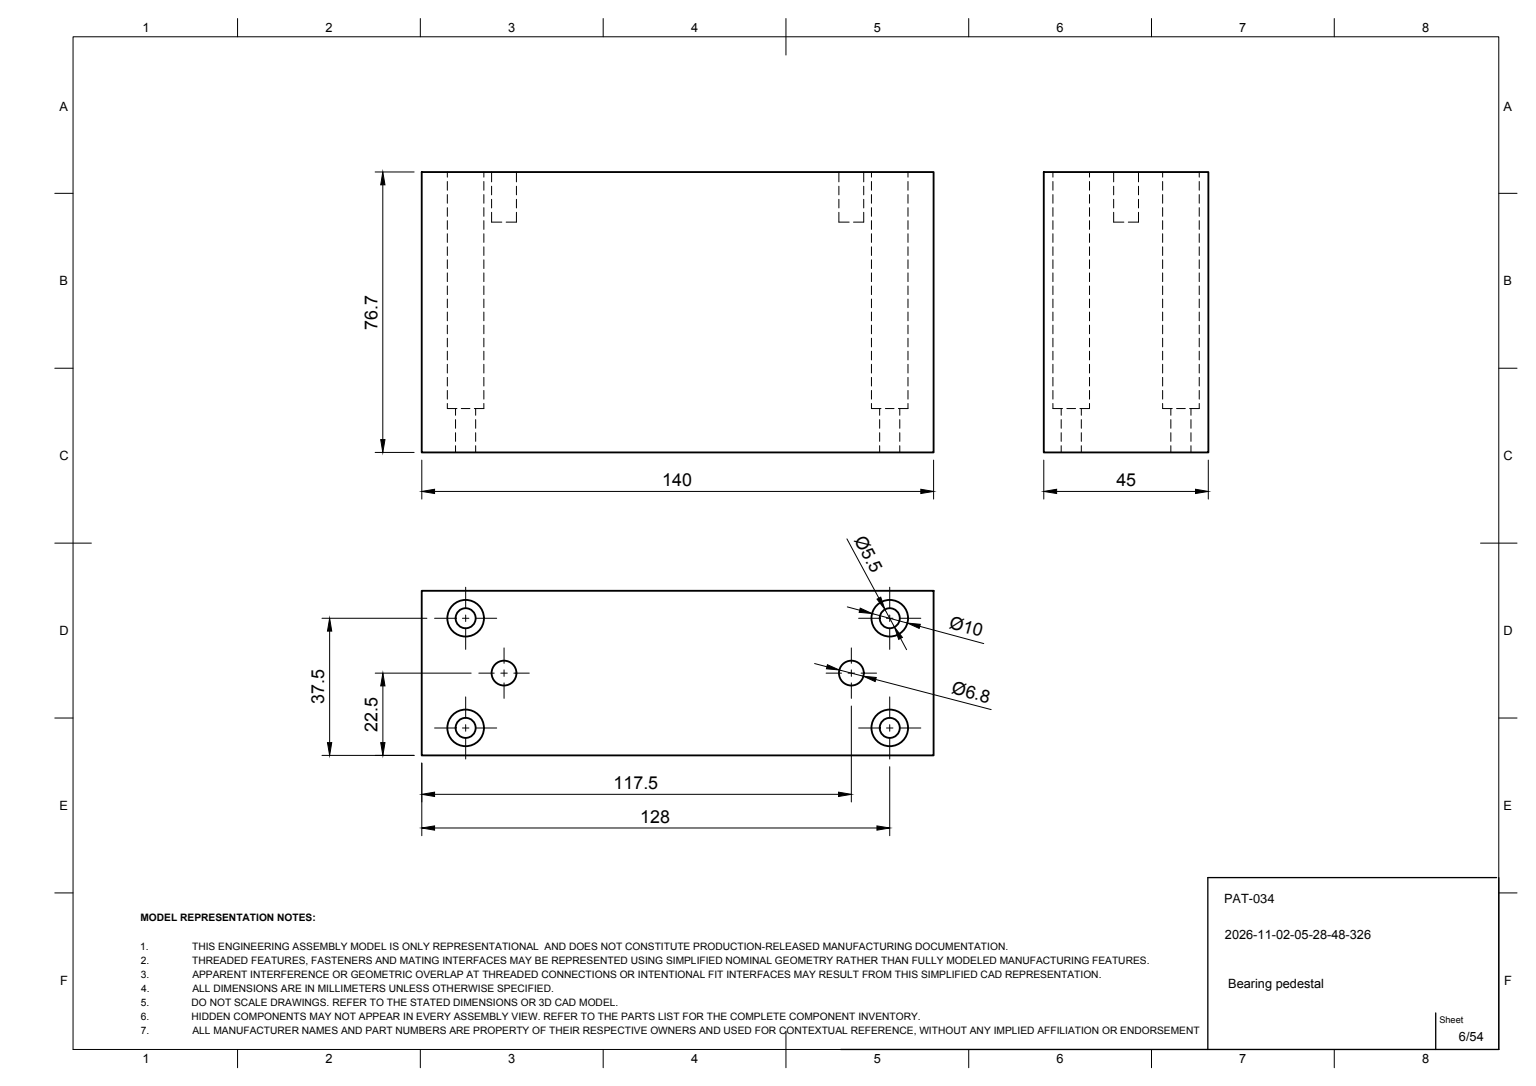
ISO-10303-21;
HEADER;
/* Generated by software containing ST-Developer
 * from STEP Tools, Inc. (www.steptools.com) 
 */

FILE_DESCRIPTION(
/* description */ ('Fatigue rig crank-slider'),
/* implementation_level */ '2;1');

FILE_NAME(
/* name */ 'Bearing pedestal.step',
/* time_stamp */ '2026-10-28T03:24:50-07:00',
/* author */ (''),
/* organization */ (''),
/* preprocessor_version */ 'ST-DEVELOPER v20.2',
/* originating_system */ 'Autodesk Translation Framework v15.17.0.0',
/* authorisation */ '');

FILE_SCHEMA (('AUTOMOTIVE_DESIGN { 1 0 10303 214 3 1 1 }'));
ENDSEC;

DATA;
#10=MECHANICAL_DESIGN_GEOMETRIC_PRESENTATION_REPRESENTATION('',(#588),#16911);
#488=SHAPE_REPRESENTATION_RELATIONSHIP('SRR','None',#17127,#538);
#538=ADVANCED_BREP_SHAPE_REPRESENTATION('',(#647),#16856);
#588=STYLED_ITEM('',(#17487),#647);
#647=MANIFOLD_SOLID_BREP('Body1',#8879);
#724=FACE_BOUND('',#1788,.T.);
#725=FACE_BOUND('',#1791,.T.);
#726=FACE_BOUND('',#1794,.T.);
#727=FACE_BOUND('',#1797,.T.);
#728=FACE_BOUND('',#1807,.T.);
#729=FACE_BOUND('',#1808,.T.);
#730=FACE_BOUND('',#1809,.T.);
#731=FACE_BOUND('',#1810,.T.);
#732=FACE_BOUND('',#1811,.T.);
#733=FACE_BOUND('',#1812,.T.);
#734=FACE_BOUND('',#1814,.T.);
#735=FACE_BOUND('',#1815,.T.);
#736=FACE_BOUND('',#1816,.T.);
#737=FACE_BOUND('',#1817,.T.);
#903=PLANE('',#9542);
#904=PLANE('',#9546);
#905=PLANE('',#9550);
#906=PLANE('',#9555);
#907=PLANE('',#9560);
#908=PLANE('',#9565);
#909=PLANE('',#9575);
#910=PLANE('',#9576);
#911=PLANE('',#9577);
#912=PLANE('',#9578);
#913=PLANE('',#9579);
#914=PLANE('',#9580);
#1235=FACE_OUTER_BOUND('',#1782,.T.);
#1236=FACE_OUTER_BOUND('',#1783,.T.);
#1237=FACE_OUTER_BOUND('',#1784,.T.);
#1238=FACE_OUTER_BOUND('',#1785,.T.);
#1239=FACE_OUTER_BOUND('',#1786,.T.);
#1240=FACE_OUTER_BOUND('',#1787,.T.);
#1241=FACE_OUTER_BOUND('',#1789,.T.);
#1242=FACE_OUTER_BOUND('',#1790,.T.);
#1243=FACE_OUTER_BOUND('',#1792,.T.);
#1244=FACE_OUTER_BOUND('',#1793,.T.);
#1245=FACE_OUTER_BOUND('',#1795,.T.);
#1246=FACE_OUTER_BOUND('',#1796,.T.);
#1247=FACE_OUTER_BOUND('',#1798,.T.);
#1248=FACE_OUTER_BOUND('',#1799,.T.);
#1249=FACE_OUTER_BOUND('',#1800,.T.);
#1250=FACE_OUTER_BOUND('',#1801,.T.);
#1251=FACE_OUTER_BOUND('',#1802,.T.);
#1252=FACE_OUTER_BOUND('',#1803,.T.);
#1253=FACE_OUTER_BOUND('',#1804,.T.);
#1254=FACE_OUTER_BOUND('',#1805,.T.);
#1255=FACE_OUTER_BOUND('',#1806,.T.);
#1256=FACE_OUTER_BOUND('',#1813,.T.);
#1782=EDGE_LOOP('',(#6092,#6093,#6094,#6095));
#1783=EDGE_LOOP('',(#6096));
#1784=EDGE_LOOP('',(#6097,#6098,#6099,#6100));
#1785=EDGE_LOOP('',(#6101));
#1786=EDGE_LOOP('',(#6102,#6103,#6104,#6105));
#1787=EDGE_LOOP('',(#6106));
#1788=EDGE_LOOP('',(#6107));
#1789=EDGE_LOOP('',(#6108,#6109,#6110,#6111));
#1790=EDGE_LOOP('',(#6112));
#1791=EDGE_LOOP('',(#6113));
#1792=EDGE_LOOP('',(#6114,#6115,#6116,#6117));
#1793=EDGE_LOOP('',(#6118));
#1794=EDGE_LOOP('',(#6119));
#1795=EDGE_LOOP('',(#6120,#6121,#6122,#6123));
#1796=EDGE_LOOP('',(#6124));
#1797=EDGE_LOOP('',(#6125));
#1798=EDGE_LOOP('',(#6126,#6127,#6128,#6129));
#1799=EDGE_LOOP('',(#6130,#6131,#6132,#6133));
#1800=EDGE_LOOP('',(#6134,#6135,#6136,#6137));
#1801=EDGE_LOOP('',(#6138,#6139,#6140,#6141));
#1802=EDGE_LOOP('',(#6142,#6143,#6144,#6145));
#1803=EDGE_LOOP('',(#6146,#6147,#6148,#6149));
#1804=EDGE_LOOP('',(#6150,#6151,#6152,#6153));
#1805=EDGE_LOOP('',(#6154,#6155,#6156,#6157));
#1806=EDGE_LOOP('',(#6158,#6159,#6160,#6161));
#1807=EDGE_LOOP('',(#6162));
#1808=EDGE_LOOP('',(#6163));
#1809=EDGE_LOOP('',(#6164));
#1810=EDGE_LOOP('',(#6165));
#1811=EDGE_LOOP('',(#6166));
#1812=EDGE_LOOP('',(#6167));
#1813=EDGE_LOOP('',(#6168,#6169,#6170,#6171));
#1814=EDGE_LOOP('',(#6172));
#1815=EDGE_LOOP('',(#6173));
#1816=EDGE_LOOP('',(#6174));
#1817=EDGE_LOOP('',(#6175));
#2484=LINE('',#13464,#3130);
#2485=LINE('',#13471,#3131);
#2486=LINE('',#13478,#3132);
#2487=LINE('',#13487,#3133);
#2488=LINE('',#13496,#3134);
#2489=LINE('',#13505,#3135);
#2490=LINE('',#13513,#3136);
#2491=LINE('',#13517,#3137);
#2492=LINE('',#13521,#3138);
#2493=LINE('',#13525,#3139);
#2494=LINE('',#13529,#3140);
#2495=LINE('',#13531,#3141);
#2496=LINE('',#13533,#3142);
#2497=LINE('',#13534,#3143);
#2498=LINE('',#13537,#3144);
#2499=LINE('',#13539,#3145);
#2500=LINE('',#13540,#3146);
#2501=LINE('',#13543,#3147);
#2502=LINE('',#13545,#3148);
#2503=LINE('',#13546,#3149);
#2504=LINE('',#13548,#3150);
#2505=LINE('',#13549,#3151);
#3130=VECTOR('',#10686,0.34);
#3131=VECTOR('',#10695,0.34);
#3132=VECTOR('',#10704,0.5);
#3133=VECTOR('',#10715,0.5);
#3134=VECTOR('',#10726,0.5);
#3135=VECTOR('',#10737,0.5);
#3136=VECTOR('',#10748,0.275);
#3137=VECTOR('',#10753,0.275);
#3138=VECTOR('',#10758,0.275);
#3139=VECTOR('',#10763,0.275);
#3140=VECTOR('',#10766,1.);
#3141=VECTOR('',#10767,1.);
#3142=VECTOR('',#10768,1.);
#3143=VECTOR('',#10769,1.);
#3144=VECTOR('',#10772,1.);
#3145=VECTOR('',#10773,1.);
#3146=VECTOR('',#10774,1.);
#3147=VECTOR('',#10777,1.);
#3148=VECTOR('',#10778,1.);
#3149=VECTOR('',#10779,1.);
#3150=VECTOR('',#10782,1.);
#3151=VECTOR('',#10783,1.);
#3776=CIRCLE('',#9540,0.34);
#3777=CIRCLE('',#9541,0.34);
#3778=CIRCLE('',#9544,0.34);
#3779=CIRCLE('',#9545,0.34);
#3780=CIRCLE('',#9548,0.5);
#3781=CIRCLE('',#9549,0.5);
#3782=CIRCLE('',#9551,0.275);
#3783=CIRCLE('',#9553,0.5);
#3784=CIRCLE('',#9554,0.5);
#3785=CIRCLE('',#9556,0.275);
#3786=CIRCLE('',#9558,0.5);
#3787=CIRCLE('',#9559,0.5);
#3788=CIRCLE('',#9561,0.275);
#3789=CIRCLE('',#9563,0.5);
#3790=CIRCLE('',#9564,0.5);
#3791=CIRCLE('',#9566,0.275);
#3792=CIRCLE('',#9568,0.275);
#3793=CIRCLE('',#9570,0.275);
#3794=CIRCLE('',#9572,0.275);
#3795=CIRCLE('',#9574,0.275);
#4184=VERTEX_POINT('',#13461);
#4185=VERTEX_POINT('',#13463);
#4186=VERTEX_POINT('',#13468);
#4187=VERTEX_POINT('',#13470);
#4188=VERTEX_POINT('',#13475);
#4189=VERTEX_POINT('',#13477);
#4190=VERTEX_POINT('',#13481);
#4191=VERTEX_POINT('',#13484);
#4192=VERTEX_POINT('',#13486);
#4193=VERTEX_POINT('',#13490);
#4194=VERTEX_POINT('',#13493);
#4195=VERTEX_POINT('',#13495);
#4196=VERTEX_POINT('',#13499);
#4197=VERTEX_POINT('',#13502);
#4198=VERTEX_POINT('',#13504);
#4199=VERTEX_POINT('',#13508);
#4200=VERTEX_POINT('',#13511);
#4201=VERTEX_POINT('',#13515);
#4202=VERTEX_POINT('',#13519);
#4203=VERTEX_POINT('',#13523);
#4204=VERTEX_POINT('',#13527);
#4205=VERTEX_POINT('',#13528);
#4206=VERTEX_POINT('',#13530);
#4207=VERTEX_POINT('',#13532);
#4208=VERTEX_POINT('',#13536);
#4209=VERTEX_POINT('',#13538);
#4210=VERTEX_POINT('',#13542);
#4211=VERTEX_POINT('',#13544);
#4944=EDGE_CURVE('',#4184,#4184,#3776,.T.);
#4945=EDGE_CURVE('',#4184,#4185,#2484,.T.);
#4946=EDGE_CURVE('',#4185,#4185,#3777,.T.);
#4947=EDGE_CURVE('',#4186,#4186,#3778,.T.);
#4948=EDGE_CURVE('',#4186,#4187,#2485,.T.);
#4949=EDGE_CURVE('',#4187,#4187,#3779,.T.);
#4950=EDGE_CURVE('',#4188,#4188,#3780,.T.);
#4951=EDGE_CURVE('',#4188,#4189,#2486,.T.);
#4952=EDGE_CURVE('',#4189,#4189,#3781,.T.);
#4953=EDGE_CURVE('',#4190,#4190,#3782,.T.);
#4954=EDGE_CURVE('',#4191,#4191,#3783,.T.);
#4955=EDGE_CURVE('',#4191,#4192,#2487,.T.);
#4956=EDGE_CURVE('',#4192,#4192,#3784,.T.);
#4957=EDGE_CURVE('',#4193,#4193,#3785,.T.);
#4958=EDGE_CURVE('',#4194,#4194,#3786,.T.);
#4959=EDGE_CURVE('',#4194,#4195,#2488,.T.);
#4960=EDGE_CURVE('',#4195,#4195,#3787,.T.);
#4961=EDGE_CURVE('',#4196,#4196,#3788,.T.);
#4962=EDGE_CURVE('',#4197,#4197,#3789,.T.);
#4963=EDGE_CURVE('',#4197,#4198,#2489,.T.);
#4964=EDGE_CURVE('',#4198,#4198,#3790,.T.);
#4965=EDGE_CURVE('',#4199,#4199,#3791,.T.);
#4966=EDGE_CURVE('',#4200,#4200,#3792,.T.);
#4967=EDGE_CURVE('',#4200,#4190,#2490,.T.);
#4968=EDGE_CURVE('',#4201,#4201,#3793,.T.);
#4969=EDGE_CURVE('',#4201,#4193,#2491,.T.);
#4970=EDGE_CURVE('',#4202,#4202,#3794,.T.);
#4971=EDGE_CURVE('',#4202,#4196,#2492,.T.);
#4972=EDGE_CURVE('',#4203,#4203,#3795,.T.);
#4973=EDGE_CURVE('',#4203,#4199,#2493,.T.);
#4974=EDGE_CURVE('',#4204,#4205,#2494,.T.);
#4975=EDGE_CURVE('',#4205,#4206,#2495,.T.);
#4976=EDGE_CURVE('',#4207,#4206,#2496,.T.);
#4977=EDGE_CURVE('',#4204,#4207,#2497,.T.);
#4978=EDGE_CURVE('',#4208,#4204,#2498,.T.);
#4979=EDGE_CURVE('',#4209,#4207,#2499,.T.);
#4980=EDGE_CURVE('',#4208,#4209,#2500,.T.);
#4981=EDGE_CURVE('',#4210,#4208,#2501,.T.);
#4982=EDGE_CURVE('',#4211,#4209,#2502,.T.);
#4983=EDGE_CURVE('',#4210,#4211,#2503,.T.);
#4984=EDGE_CURVE('',#4205,#4210,#2504,.T.);
#4985=EDGE_CURVE('',#4206,#4211,#2505,.T.);
#6092=ORIENTED_EDGE('',*,*,#4944,.F.);
#6093=ORIENTED_EDGE('',*,*,#4945,.T.);
#6094=ORIENTED_EDGE('',*,*,#4946,.F.);
#6095=ORIENTED_EDGE('',*,*,#4945,.F.);
#6096=ORIENTED_EDGE('',*,*,#4944,.T.);
#6097=ORIENTED_EDGE('',*,*,#4947,.F.);
#6098=ORIENTED_EDGE('',*,*,#4948,.T.);
#6099=ORIENTED_EDGE('',*,*,#4949,.F.);
#6100=ORIENTED_EDGE('',*,*,#4948,.F.);
#6101=ORIENTED_EDGE('',*,*,#4947,.T.);
#6102=ORIENTED_EDGE('',*,*,#4950,.F.);
#6103=ORIENTED_EDGE('',*,*,#4951,.T.);
#6104=ORIENTED_EDGE('',*,*,#4952,.F.);
#6105=ORIENTED_EDGE('',*,*,#4951,.F.);
#6106=ORIENTED_EDGE('',*,*,#4950,.T.);
#6107=ORIENTED_EDGE('',*,*,#4953,.F.);
#6108=ORIENTED_EDGE('',*,*,#4954,.F.);
#6109=ORIENTED_EDGE('',*,*,#4955,.T.);
#6110=ORIENTED_EDGE('',*,*,#4956,.F.);
#6111=ORIENTED_EDGE('',*,*,#4955,.F.);
#6112=ORIENTED_EDGE('',*,*,#4954,.T.);
#6113=ORIENTED_EDGE('',*,*,#4957,.F.);
#6114=ORIENTED_EDGE('',*,*,#4958,.F.);
#6115=ORIENTED_EDGE('',*,*,#4959,.T.);
#6116=ORIENTED_EDGE('',*,*,#4960,.F.);
#6117=ORIENTED_EDGE('',*,*,#4959,.F.);
#6118=ORIENTED_EDGE('',*,*,#4958,.T.);
#6119=ORIENTED_EDGE('',*,*,#4961,.F.);
#6120=ORIENTED_EDGE('',*,*,#4962,.F.);
#6121=ORIENTED_EDGE('',*,*,#4963,.T.);
#6122=ORIENTED_EDGE('',*,*,#4964,.F.);
#6123=ORIENTED_EDGE('',*,*,#4963,.F.);
#6124=ORIENTED_EDGE('',*,*,#4962,.T.);
#6125=ORIENTED_EDGE('',*,*,#4965,.F.);
#6126=ORIENTED_EDGE('',*,*,#4966,.F.);
#6127=ORIENTED_EDGE('',*,*,#4967,.T.);
#6128=ORIENTED_EDGE('',*,*,#4953,.T.);
#6129=ORIENTED_EDGE('',*,*,#4967,.F.);
#6130=ORIENTED_EDGE('',*,*,#4968,.F.);
#6131=ORIENTED_EDGE('',*,*,#4969,.T.);
#6132=ORIENTED_EDGE('',*,*,#4957,.T.);
#6133=ORIENTED_EDGE('',*,*,#4969,.F.);
#6134=ORIENTED_EDGE('',*,*,#4970,.F.);
#6135=ORIENTED_EDGE('',*,*,#4971,.T.);
#6136=ORIENTED_EDGE('',*,*,#4961,.T.);
#6137=ORIENTED_EDGE('',*,*,#4971,.F.);
#6138=ORIENTED_EDGE('',*,*,#4972,.F.);
#6139=ORIENTED_EDGE('',*,*,#4973,.T.);
#6140=ORIENTED_EDGE('',*,*,#4965,.T.);
#6141=ORIENTED_EDGE('',*,*,#4973,.F.);
#6142=ORIENTED_EDGE('',*,*,#4974,.T.);
#6143=ORIENTED_EDGE('',*,*,#4975,.T.);
#6144=ORIENTED_EDGE('',*,*,#4976,.F.);
#6145=ORIENTED_EDGE('',*,*,#4977,.F.);
#6146=ORIENTED_EDGE('',*,*,#4978,.T.);
#6147=ORIENTED_EDGE('',*,*,#4977,.T.);
#6148=ORIENTED_EDGE('',*,*,#4979,.F.);
#6149=ORIENTED_EDGE('',*,*,#4980,.F.);
#6150=ORIENTED_EDGE('',*,*,#4981,.T.);
#6151=ORIENTED_EDGE('',*,*,#4980,.T.);
#6152=ORIENTED_EDGE('',*,*,#4982,.F.);
#6153=ORIENTED_EDGE('',*,*,#4983,.F.);
#6154=ORIENTED_EDGE('',*,*,#4984,.T.);
#6155=ORIENTED_EDGE('',*,*,#4983,.T.);
#6156=ORIENTED_EDGE('',*,*,#4985,.F.);
#6157=ORIENTED_EDGE('',*,*,#4975,.F.);
#6158=ORIENTED_EDGE('',*,*,#4985,.T.);
#6159=ORIENTED_EDGE('',*,*,#4982,.T.);
#6160=ORIENTED_EDGE('',*,*,#4979,.T.);
#6161=ORIENTED_EDGE('',*,*,#4976,.T.);
#6162=ORIENTED_EDGE('',*,*,#4946,.T.);
#6163=ORIENTED_EDGE('',*,*,#4949,.T.);
#6164=ORIENTED_EDGE('',*,*,#4964,.T.);
#6165=ORIENTED_EDGE('',*,*,#4960,.T.);
#6166=ORIENTED_EDGE('',*,*,#4956,.T.);
#6167=ORIENTED_EDGE('',*,*,#4952,.T.);
#6168=ORIENTED_EDGE('',*,*,#4984,.F.);
#6169=ORIENTED_EDGE('',*,*,#4974,.F.);
#6170=ORIENTED_EDGE('',*,*,#4978,.F.);
#6171=ORIENTED_EDGE('',*,*,#4981,.F.);
#6172=ORIENTED_EDGE('',*,*,#4966,.T.);
#6173=ORIENTED_EDGE('',*,*,#4968,.T.);
#6174=ORIENTED_EDGE('',*,*,#4970,.T.);
#6175=ORIENTED_EDGE('',*,*,#4972,.T.);
#8208=CYLINDRICAL_SURFACE('',#9539,0.34);
#8209=CYLINDRICAL_SURFACE('',#9543,0.34);
#8210=CYLINDRICAL_SURFACE('',#9547,0.5);
#8211=CYLINDRICAL_SURFACE('',#9552,0.5);
#8212=CYLINDRICAL_SURFACE('',#9557,0.5);
#8213=CYLINDRICAL_SURFACE('',#9562,0.5);
#8214=CYLINDRICAL_SURFACE('',#9567,0.275);
#8215=CYLINDRICAL_SURFACE('',#9569,0.275);
#8216=CYLINDRICAL_SURFACE('',#9571,0.275);
#8217=CYLINDRICAL_SURFACE('',#9573,0.275);
#8373=ADVANCED_FACE('',(#1235),#8208,.F.);
#8374=ADVANCED_FACE('',(#1236),#903,.T.);
#8375=ADVANCED_FACE('',(#1237),#8209,.F.);
#8376=ADVANCED_FACE('',(#1238),#904,.T.);
#8377=ADVANCED_FACE('',(#1239),#8210,.F.);
#8378=ADVANCED_FACE('',(#1240,#724),#905,.T.);
#8379=ADVANCED_FACE('',(#1241),#8211,.F.);
#8380=ADVANCED_FACE('',(#1242,#725),#906,.T.);
#8381=ADVANCED_FACE('',(#1243),#8212,.F.);
#8382=ADVANCED_FACE('',(#1244,#726),#907,.T.);
#8383=ADVANCED_FACE('',(#1245),#8213,.F.);
#8384=ADVANCED_FACE('',(#1246,#727),#908,.T.);
#8385=ADVANCED_FACE('',(#1247),#8214,.F.);
#8386=ADVANCED_FACE('',(#1248),#8215,.F.);
#8387=ADVANCED_FACE('',(#1249),#8216,.F.);
#8388=ADVANCED_FACE('',(#1250),#8217,.F.);
#8389=ADVANCED_FACE('',(#1251),#909,.T.);
#8390=ADVANCED_FACE('',(#1252),#910,.T.);
#8391=ADVANCED_FACE('',(#1253),#911,.T.);
#8392=ADVANCED_FACE('',(#1254),#912,.T.);
#8393=ADVANCED_FACE('',(#1255,#728,#729,#730,#731,#732,#733),#913,.T.);
#8394=ADVANCED_FACE('',(#1256,#734,#735,#736,#737),#914,.F.);
#8879=CLOSED_SHELL('',(#8373,#8374,#8375,#8376,#8377,#8378,#8379,#8380,
#8381,#8382,#8383,#8384,#8385,#8386,#8387,#8388,#8389,#8390,#8391,#8392,
#8393,#8394));
#9538=AXIS2_PLACEMENT_3D('',#13459,#10680,#10681);
#9539=AXIS2_PLACEMENT_3D('',#13460,#10682,#10683);
#9540=AXIS2_PLACEMENT_3D('',#13462,#10684,#10685);
#9541=AXIS2_PLACEMENT_3D('',#13465,#10687,#10688);
#9542=AXIS2_PLACEMENT_3D('',#13466,#10689,#10690);
#9543=AXIS2_PLACEMENT_3D('',#13467,#10691,#10692);
#9544=AXIS2_PLACEMENT_3D('',#13469,#10693,#10694);
#9545=AXIS2_PLACEMENT_3D('',#13472,#10696,#10697);
#9546=AXIS2_PLACEMENT_3D('',#13473,#10698,#10699);
#9547=AXIS2_PLACEMENT_3D('',#13474,#10700,#10701);
#9548=AXIS2_PLACEMENT_3D('',#13476,#10702,#10703);
#9549=AXIS2_PLACEMENT_3D('',#13479,#10705,#10706);
#9550=AXIS2_PLACEMENT_3D('',#13480,#10707,#10708);
#9551=AXIS2_PLACEMENT_3D('',#13482,#10709,#10710);
#9552=AXIS2_PLACEMENT_3D('',#13483,#10711,#10712);
#9553=AXIS2_PLACEMENT_3D('',#13485,#10713,#10714);
#9554=AXIS2_PLACEMENT_3D('',#13488,#10716,#10717);
#9555=AXIS2_PLACEMENT_3D('',#13489,#10718,#10719);
#9556=AXIS2_PLACEMENT_3D('',#13491,#10720,#10721);
#9557=AXIS2_PLACEMENT_3D('',#13492,#10722,#10723);
#9558=AXIS2_PLACEMENT_3D('',#13494,#10724,#10725);
#9559=AXIS2_PLACEMENT_3D('',#13497,#10727,#10728);
#9560=AXIS2_PLACEMENT_3D('',#13498,#10729,#10730);
#9561=AXIS2_PLACEMENT_3D('',#13500,#10731,#10732);
#9562=AXIS2_PLACEMENT_3D('',#13501,#10733,#10734);
#9563=AXIS2_PLACEMENT_3D('',#13503,#10735,#10736);
#9564=AXIS2_PLACEMENT_3D('',#13506,#10738,#10739);
#9565=AXIS2_PLACEMENT_3D('',#13507,#10740,#10741);
#9566=AXIS2_PLACEMENT_3D('',#13509,#10742,#10743);
#9567=AXIS2_PLACEMENT_3D('',#13510,#10744,#10745);
#9568=AXIS2_PLACEMENT_3D('',#13512,#10746,#10747);
#9569=AXIS2_PLACEMENT_3D('',#13514,#10749,#10750);
#9570=AXIS2_PLACEMENT_3D('',#13516,#10751,#10752);
#9571=AXIS2_PLACEMENT_3D('',#13518,#10754,#10755);
#9572=AXIS2_PLACEMENT_3D('',#13520,#10756,#10757);
#9573=AXIS2_PLACEMENT_3D('',#13522,#10759,#10760);
#9574=AXIS2_PLACEMENT_3D('',#13524,#10761,#10762);
#9575=AXIS2_PLACEMENT_3D('',#13526,#10764,#10765);
#9576=AXIS2_PLACEMENT_3D('',#13535,#10770,#10771);
#9577=AXIS2_PLACEMENT_3D('',#13541,#10775,#10776);
#9578=AXIS2_PLACEMENT_3D('',#13547,#10780,#10781);
#9579=AXIS2_PLACEMENT_3D('',#13550,#10784,#10785);
#9580=AXIS2_PLACEMENT_3D('',#13551,#10786,#10787);
#10680=DIRECTION('axis',(0.,0.,1.));
#10681=DIRECTION('refdir',(1.,0.,0.));
#10682=DIRECTION('center_axis',(0.,0.,1.));
#10683=DIRECTION('ref_axis',(1.,0.,0.));
#10684=DIRECTION('center_axis',(0.,0.,1.));
#10685=DIRECTION('ref_axis',(1.,0.,0.));
#10686=DIRECTION('',(0.,0.,1.));
#10687=DIRECTION('center_axis',(0.,0.,-1.));
#10688=DIRECTION('ref_axis',(1.,0.,0.));
#10689=DIRECTION('center_axis',(0.,0.,1.));
#10690=DIRECTION('ref_axis',(1.,0.,0.));
#10691=DIRECTION('center_axis',(0.,0.,1.));
#10692=DIRECTION('ref_axis',(1.,0.,0.));
#10693=DIRECTION('center_axis',(0.,0.,1.));
#10694=DIRECTION('ref_axis',(1.,0.,0.));
#10695=DIRECTION('',(0.,0.,1.));
#10696=DIRECTION('center_axis',(0.,0.,-1.));
#10697=DIRECTION('ref_axis',(1.,0.,0.));
#10698=DIRECTION('center_axis',(0.,0.,1.));
#10699=DIRECTION('ref_axis',(1.,0.,0.));
#10700=DIRECTION('center_axis',(0.,0.,1.));
#10701=DIRECTION('ref_axis',(1.,0.,0.));
#10702=DIRECTION('center_axis',(0.,0.,1.));
#10703=DIRECTION('ref_axis',(1.,0.,0.));
#10704=DIRECTION('',(0.,0.,1.));
#10705=DIRECTION('center_axis',(0.,0.,-1.));
#10706=DIRECTION('ref_axis',(1.,0.,0.));
#10707=DIRECTION('center_axis',(0.,0.,1.));
#10708=DIRECTION('ref_axis',(1.,0.,0.));
#10709=DIRECTION('center_axis',(0.,0.,1.));
#10710=DIRECTION('ref_axis',(1.,0.,0.));
#10711=DIRECTION('center_axis',(0.,0.,1.));
#10712=DIRECTION('ref_axis',(1.,0.,0.));
#10713=DIRECTION('center_axis',(0.,0.,1.));
#10714=DIRECTION('ref_axis',(1.,0.,0.));
#10715=DIRECTION('',(0.,0.,1.));
#10716=DIRECTION('center_axis',(0.,0.,-1.));
#10717=DIRECTION('ref_axis',(1.,0.,0.));
#10718=DIRECTION('center_axis',(0.,0.,1.));
#10719=DIRECTION('ref_axis',(1.,0.,0.));
#10720=DIRECTION('center_axis',(0.,0.,1.));
#10721=DIRECTION('ref_axis',(1.,0.,0.));
#10722=DIRECTION('center_axis',(0.,0.,1.));
#10723=DIRECTION('ref_axis',(1.,0.,0.));
#10724=DIRECTION('center_axis',(0.,0.,1.));
#10725=DIRECTION('ref_axis',(1.,0.,0.));
#10726=DIRECTION('',(0.,0.,1.));
#10727=DIRECTION('center_axis',(0.,0.,-1.));
#10728=DIRECTION('ref_axis',(1.,0.,0.));
#10729=DIRECTION('center_axis',(0.,0.,1.));
#10730=DIRECTION('ref_axis',(1.,0.,0.));
#10731=DIRECTION('center_axis',(0.,0.,1.));
#10732=DIRECTION('ref_axis',(1.,0.,0.));
#10733=DIRECTION('center_axis',(0.,0.,1.));
#10734=DIRECTION('ref_axis',(1.,0.,0.));
#10735=DIRECTION('center_axis',(0.,0.,1.));
#10736=DIRECTION('ref_axis',(1.,0.,0.));
#10737=DIRECTION('',(0.,0.,1.));
#10738=DIRECTION('center_axis',(0.,0.,-1.));
#10739=DIRECTION('ref_axis',(1.,0.,0.));
#10740=DIRECTION('center_axis',(0.,0.,1.));
#10741=DIRECTION('ref_axis',(1.,0.,0.));
#10742=DIRECTION('center_axis',(0.,0.,1.));
#10743=DIRECTION('ref_axis',(1.,0.,0.));
#10744=DIRECTION('center_axis',(0.,0.,1.));
#10745=DIRECTION('ref_axis',(1.,0.,0.));
#10746=DIRECTION('center_axis',(0.,0.,1.));
#10747=DIRECTION('ref_axis',(1.,0.,0.));
#10748=DIRECTION('',(0.,0.,1.));
#10749=DIRECTION('center_axis',(0.,0.,1.));
#10750=DIRECTION('ref_axis',(1.,0.,0.));
#10751=DIRECTION('center_axis',(0.,0.,1.));
#10752=DIRECTION('ref_axis',(1.,0.,0.));
#10753=DIRECTION('',(0.,0.,1.));
#10754=DIRECTION('center_axis',(0.,0.,1.));
#10755=DIRECTION('ref_axis',(1.,0.,0.));
#10756=DIRECTION('center_axis',(0.,0.,1.));
#10757=DIRECTION('ref_axis',(1.,0.,0.));
#10758=DIRECTION('',(0.,0.,1.));
#10759=DIRECTION('center_axis',(0.,0.,1.));
#10760=DIRECTION('ref_axis',(1.,0.,0.));
#10761=DIRECTION('center_axis',(0.,0.,1.));
#10762=DIRECTION('ref_axis',(1.,0.,0.));
#10763=DIRECTION('',(0.,0.,1.));
#10764=DIRECTION('center_axis',(0.,1.,0.));
#10765=DIRECTION('ref_axis',(-1.,0.,0.));
#10766=DIRECTION('',(-1.,0.,0.));
#10767=DIRECTION('',(0.,0.,1.));
#10768=DIRECTION('',(-1.,0.,0.));
#10769=DIRECTION('',(0.,0.,1.));
#10770=DIRECTION('center_axis',(1.,0.,0.));
#10771=DIRECTION('ref_axis',(0.,1.,0.));
#10772=DIRECTION('',(0.,1.,0.));
#10773=DIRECTION('',(0.,1.,0.));
#10774=DIRECTION('',(0.,0.,1.));
#10775=DIRECTION('center_axis',(0.,-1.,0.));
#10776=DIRECTION('ref_axis',(1.,0.,0.));
#10777=DIRECTION('',(1.,0.,0.));
#10778=DIRECTION('',(1.,0.,0.));
#10779=DIRECTION('',(0.,0.,1.));
#10780=DIRECTION('center_axis',(-1.,0.,0.));
#10781=DIRECTION('ref_axis',(0.,-1.,0.));
#10782=DIRECTION('',(0.,-1.,0.));
#10783=DIRECTION('',(0.,-1.,0.));
#10784=DIRECTION('center_axis',(0.,0.,1.));
#10785=DIRECTION('ref_axis',(1.,0.,0.));
#10786=DIRECTION('center_axis',(0.,0.,1.));
#10787=DIRECTION('ref_axis',(1.,0.,0.));
#13459=CARTESIAN_POINT('',(0.,0.,0.));
#13460=CARTESIAN_POINT('Origin',(-4.75,-15.,7.3));
#13461=CARTESIAN_POINT('',(-5.09,-15.,7.3));
#13462=CARTESIAN_POINT('Origin',(-4.75,-15.,7.3));
#13463=CARTESIAN_POINT('',(-5.09,-15.,8.67));
#13464=CARTESIAN_POINT('',(-5.09,-15.,7.3));
#13465=CARTESIAN_POINT('Origin',(-4.75,-15.,8.67));
#13466=CARTESIAN_POINT('Origin',(-4.75,-15.,7.3));
#13467=CARTESIAN_POINT('Origin',(4.75,-15.,7.3));
#13468=CARTESIAN_POINT('',(4.41,-15.,7.3));
#13469=CARTESIAN_POINT('Origin',(4.75,-15.,7.3));
#13470=CARTESIAN_POINT('',(4.41,-15.,8.67));
#13471=CARTESIAN_POINT('',(4.41,-15.,7.3));
#13472=CARTESIAN_POINT('Origin',(4.75,-15.,8.67));
#13473=CARTESIAN_POINT('Origin',(4.75,-15.,7.3));
#13474=CARTESIAN_POINT('Origin',(5.8,-16.5,2.2));
#13475=CARTESIAN_POINT('',(5.3,-16.5,2.2));
#13476=CARTESIAN_POINT('Origin',(5.8,-16.5,2.2));
#13477=CARTESIAN_POINT('',(5.3,-16.5,8.67));
#13478=CARTESIAN_POINT('',(5.3,-16.5,2.2));
#13479=CARTESIAN_POINT('Origin',(5.8,-16.5,8.67));
#13480=CARTESIAN_POINT('Origin',(5.8,-16.5,2.2));
#13481=CARTESIAN_POINT('',(5.525,-16.5,2.2));
#13482=CARTESIAN_POINT('Origin',(5.8,-16.5,2.2));
#13483=CARTESIAN_POINT('Origin',(-5.8,-13.5,2.2));
#13484=CARTESIAN_POINT('',(-6.3,-13.5,2.2));
#13485=CARTESIAN_POINT('Origin',(-5.8,-13.5,2.2));
#13486=CARTESIAN_POINT('',(-6.3,-13.5,8.67));
#13487=CARTESIAN_POINT('',(-6.3,-13.5,2.2));
#13488=CARTESIAN_POINT('Origin',(-5.8,-13.5,8.67));
#13489=CARTESIAN_POINT('Origin',(-5.8,-13.5,2.2));
#13490=CARTESIAN_POINT('',(-6.075,-13.5,2.2));
#13491=CARTESIAN_POINT('Origin',(-5.8,-13.5,2.2));
#13492=CARTESIAN_POINT('Origin',(-5.8,-16.5,2.2));
#13493=CARTESIAN_POINT('',(-6.3,-16.5,2.2));
#13494=CARTESIAN_POINT('Origin',(-5.8,-16.5,2.2));
#13495=CARTESIAN_POINT('',(-6.3,-16.5,8.67));
#13496=CARTESIAN_POINT('',(-6.3,-16.5,2.2));
#13497=CARTESIAN_POINT('Origin',(-5.8,-16.5,8.67));
#13498=CARTESIAN_POINT('Origin',(-5.8,-16.5,2.2));
#13499=CARTESIAN_POINT('',(-6.075,-16.5,2.2));
#13500=CARTESIAN_POINT('Origin',(-5.8,-16.5,2.2));
#13501=CARTESIAN_POINT('Origin',(5.8,-13.5,2.2));
#13502=CARTESIAN_POINT('',(5.3,-13.5,2.2));
#13503=CARTESIAN_POINT('Origin',(5.8,-13.5,2.2));
#13504=CARTESIAN_POINT('',(5.3,-13.5,8.67));
#13505=CARTESIAN_POINT('',(5.3,-13.5,2.2));
#13506=CARTESIAN_POINT('Origin',(5.8,-13.5,8.67));
#13507=CARTESIAN_POINT('Origin',(5.8,-13.5,2.2));
#13508=CARTESIAN_POINT('',(5.525,-13.5,2.2));
#13509=CARTESIAN_POINT('Origin',(5.8,-13.5,2.2));
#13510=CARTESIAN_POINT('Origin',(5.8,-16.5,0.9));
#13511=CARTESIAN_POINT('',(5.525,-16.5,1.));
#13512=CARTESIAN_POINT('Origin',(5.8,-16.5,1.));
#13513=CARTESIAN_POINT('',(5.525,-16.5,0.9));
#13514=CARTESIAN_POINT('Origin',(-5.8,-13.5,0.9));
#13515=CARTESIAN_POINT('',(-6.075,-13.5,1.));
#13516=CARTESIAN_POINT('Origin',(-5.8,-13.5,1.));
#13517=CARTESIAN_POINT('',(-6.075,-13.5,0.9));
#13518=CARTESIAN_POINT('Origin',(-5.8,-16.5,0.9));
#13519=CARTESIAN_POINT('',(-6.075,-16.5,1.));
#13520=CARTESIAN_POINT('Origin',(-5.8,-16.5,1.));
#13521=CARTESIAN_POINT('',(-6.075,-16.5,0.9));
#13522=CARTESIAN_POINT('Origin',(5.8,-13.5,0.9));
#13523=CARTESIAN_POINT('',(5.525,-13.5,1.));
#13524=CARTESIAN_POINT('Origin',(5.8,-13.5,1.));
#13525=CARTESIAN_POINT('',(5.525,-13.5,0.9));
#13526=CARTESIAN_POINT('Origin',(7.,-12.75,1.));
#13527=CARTESIAN_POINT('',(7.,-12.75,1.));
#13528=CARTESIAN_POINT('',(-7.,-12.75,1.));
#13529=CARTESIAN_POINT('',(7.,-12.75,1.));
#13530=CARTESIAN_POINT('',(-7.,-12.75,8.67));
#13531=CARTESIAN_POINT('',(-7.,-12.75,1.));
#13532=CARTESIAN_POINT('',(7.,-12.75,8.67));
#13533=CARTESIAN_POINT('',(7.,-12.75,8.67));
#13534=CARTESIAN_POINT('',(7.,-12.75,1.));
#13535=CARTESIAN_POINT('Origin',(7.,-17.25,1.));
#13536=CARTESIAN_POINT('',(7.,-17.25,1.));
#13537=CARTESIAN_POINT('',(7.,-17.25,1.));
#13538=CARTESIAN_POINT('',(7.,-17.25,8.67));
#13539=CARTESIAN_POINT('',(7.,-17.25,8.67));
#13540=CARTESIAN_POINT('',(7.,-17.25,1.));
#13541=CARTESIAN_POINT('Origin',(-7.,-17.25,1.));
#13542=CARTESIAN_POINT('',(-7.,-17.25,1.));
#13543=CARTESIAN_POINT('',(-7.,-17.25,1.));
#13544=CARTESIAN_POINT('',(-7.,-17.25,8.67));
#13545=CARTESIAN_POINT('',(-7.,-17.25,8.67));
#13546=CARTESIAN_POINT('',(-7.,-17.25,1.));
#13547=CARTESIAN_POINT('Origin',(-7.,-12.75,1.));
#13548=CARTESIAN_POINT('',(-7.,-12.75,1.));
#13549=CARTESIAN_POINT('',(-7.,-12.75,8.67));
#13550=CARTESIAN_POINT('Origin',(0.,-15.,8.67));
#13551=CARTESIAN_POINT('Origin',(0.,-15.,1.));
#16797=UNCERTAINTY_MEASURE_WITH_UNIT(LENGTH_MEASURE(0.001),#16912,
'DISTANCE_ACCURACY_VALUE',
'Maximum model space distance between geometric entities at asserted c
onnectivities');
#16852=UNCERTAINTY_MEASURE_WITH_UNIT(LENGTH_MEASURE(0.001),#16912,
'DISTANCE_ACCURACY_VALUE',
'Maximum model space distance between geometric entities at asserted c
onnectivities');
#16856=(
GEOMETRIC_REPRESENTATION_CONTEXT(3)
GLOBAL_UNCERTAINTY_ASSIGNED_CONTEXT((#16797))
GLOBAL_UNIT_ASSIGNED_CONTEXT((#16912,#16914,#16915))
REPRESENTATION_CONTEXT('','3D')
);
#16911=(
GEOMETRIC_REPRESENTATION_CONTEXT(3)
GLOBAL_UNCERTAINTY_ASSIGNED_CONTEXT((#16852))
GLOBAL_UNIT_ASSIGNED_CONTEXT((#16912,#16914,#16915))
REPRESENTATION_CONTEXT('','3D')
);
#16912=(
LENGTH_UNIT()
NAMED_UNIT(*)
SI_UNIT(.CENTI.,.METRE.)
);
#16914=(
NAMED_UNIT(*)
PLANE_ANGLE_UNIT()
SI_UNIT($,.RADIAN.)
);
#16915=(
NAMED_UNIT(*)
SI_UNIT($,.STERADIAN.)
SOLID_ANGLE_UNIT()
);
#16919=SHAPE_DEFINITION_REPRESENTATION(#16977,#17127);
#16977=PRODUCT_DEFINITION_SHAPE('',$,#17186);
#17127=SHAPE_REPRESENTATION('',(#9538),#16856);
#17182=PRODUCT_DEFINITION_CONTEXT('part definition',#17358,'design');
#17186=PRODUCT_DEFINITION('Bearing pedestal','Bearing pedestal',#17244,
#17182);
#17244=PRODUCT_DEFINITION_FORMATION('',$,#17363);
#17358=APPLICATION_CONTEXT(
'Core Data for Automotive Mechanical Design Process');
#17359=PRODUCT_CONTEXT('part definition',#17358,'mechanical');
#17363=PRODUCT('Bearing pedestal','Bearing pedestal','Bearing pedestal',
(#17359));
#17481=COLOUR_RGB('Grey',0.48,0.52,0.57);
#17482=FILL_AREA_STYLE_COLOUR('',#17481);
#17483=FILL_AREA_STYLE('',(#17482));
#17484=SURFACE_STYLE_FILL_AREA(#17483);
#17485=SURFACE_SIDE_STYLE('',(#17484));
#17486=SURFACE_STYLE_USAGE(.BOTH.,#17485);
#17487=PRESENTATION_STYLE_ASSIGNMENT((#17486));
ENDSEC;
END-ISO-10303-21;
